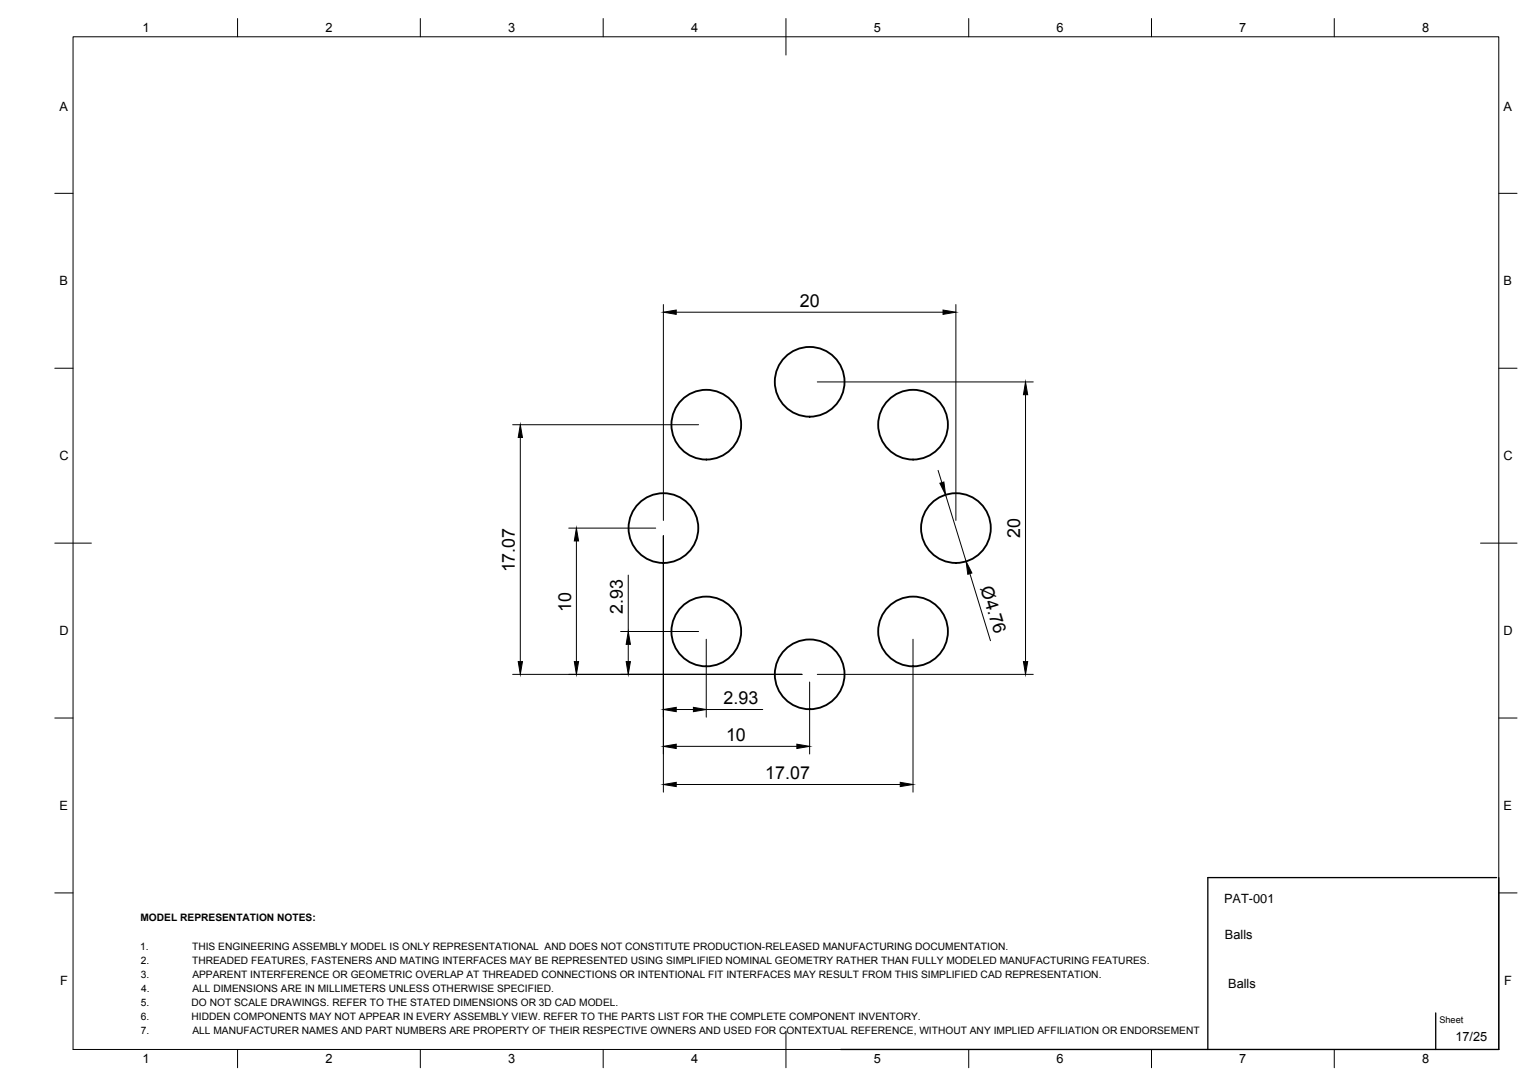
ISO-10303-21;
HEADER;
/* Generated by software containing ST-Developer
 * from STEP Tools, Inc. (www.steptools.com) 
 */

FILE_DESCRIPTION(
/* description */ ('PAT-001'),
/* implementation_level */ '2;1');

FILE_NAME(
/* name */ 'Balls.step',
/* time_stamp */ '2026-10-29T17:07:15-07:00',
/* author */ (''),
/* organization */ (''),
/* preprocessor_version */ 'ST-DEVELOPER v20.2',
/* originating_system */ 'Autodesk Translation Framework v15.17.0.0',
/* authorisation */ '');

FILE_SCHEMA (('AUTOMOTIVE_DESIGN { 1 0 10303 214 3 1 1 }'));
ENDSEC;

DATA;
#10=MECHANICAL_DESIGN_GEOMETRIC_PRESENTATION_REPRESENTATION('',(#380,#381,#382,#383,#384,#385,#386,#387),#9622);
#289=SPHERICAL_SURFACE('',#5611,0.23815);
#290=SPHERICAL_SURFACE('',#5613,0.23815);
#291=SPHERICAL_SURFACE('',#5615,0.23815);
#292=SPHERICAL_SURFACE('',#5617,0.23815);
#293=SPHERICAL_SURFACE('',#5619,0.23815);
#294=SPHERICAL_SURFACE('',#5621,0.23815);
#295=SPHERICAL_SURFACE('',#5623,0.23815);
#296=SPHERICAL_SURFACE('',#5625,0.23815);
#330=SHAPE_REPRESENTATION_RELATIONSHIP('SRR','None',#9754,#355);
#355=ADVANCED_BREP_SHAPE_REPRESENTATION('',(#413,#414,#415,#416,#417,#418,
#419,#420),#9603);
#380=STYLED_ITEM('',(#9962),#413);
#381=STYLED_ITEM('',(#9962),#414);
#382=STYLED_ITEM('',(#9962),#415);
#383=STYLED_ITEM('',(#9962),#416);
#384=STYLED_ITEM('',(#9962),#417);
#385=STYLED_ITEM('',(#9962),#418);
#386=STYLED_ITEM('',(#9962),#419);
#387=STYLED_ITEM('',(#9962),#420);
#413=MANIFOLD_SOLID_BREP('Body1',#5205);
#414=MANIFOLD_SOLID_BREP('Body2',#5206);
#415=MANIFOLD_SOLID_BREP('Body3',#5207);
#416=MANIFOLD_SOLID_BREP('Body4',#5208);
#417=MANIFOLD_SOLID_BREP('Body5',#5209);
#418=MANIFOLD_SOLID_BREP('Body6',#5210);
#419=MANIFOLD_SOLID_BREP('Body7',#5211);
#420=MANIFOLD_SOLID_BREP('Body8',#5212);
#758=FACE_OUTER_BOUND('',#1070,.T.);
#759=FACE_OUTER_BOUND('',#1071,.T.);
#760=FACE_OUTER_BOUND('',#1072,.T.);
#761=FACE_OUTER_BOUND('',#1073,.T.);
#762=FACE_OUTER_BOUND('',#1074,.T.);
#763=FACE_OUTER_BOUND('',#1075,.T.);
#764=FACE_OUTER_BOUND('',#1076,.T.);
#765=FACE_OUTER_BOUND('',#1077,.T.);
#1070=EDGE_LOOP('',(#3659,#3660));
#1071=EDGE_LOOP('',(#3661,#3662));
#1072=EDGE_LOOP('',(#3663,#3664));
#1073=EDGE_LOOP('',(#3665,#3666));
#1074=EDGE_LOOP('',(#3667,#3668));
#1075=EDGE_LOOP('',(#3669,#3670));
#1076=EDGE_LOOP('',(#3671,#3672));
#1077=EDGE_LOOP('',(#3673,#3674));
#2256=CIRCLE('',#5612,0.23815);
#2257=CIRCLE('',#5614,0.23815);
#2258=CIRCLE('',#5616,0.23815);
#2259=CIRCLE('',#5618,0.23815);
#2260=CIRCLE('',#5620,0.23815);
#2261=CIRCLE('',#5622,0.23815);
#2262=CIRCLE('',#5624,0.23815);
#2263=CIRCLE('',#5626,0.23815);
#2466=VERTEX_POINT('',#7880);
#2467=VERTEX_POINT('',#7881);
#2468=VERTEX_POINT('',#7884);
#2469=VERTEX_POINT('',#7885);
#2470=VERTEX_POINT('',#7888);
#2471=VERTEX_POINT('',#7889);
#2472=VERTEX_POINT('',#7892);
#2473=VERTEX_POINT('',#7893);
#2474=VERTEX_POINT('',#7896);
#2475=VERTEX_POINT('',#7897);
#2476=VERTEX_POINT('',#7900);
#2477=VERTEX_POINT('',#7901);
#2478=VERTEX_POINT('',#7904);
#2479=VERTEX_POINT('',#7905);
#2480=VERTEX_POINT('',#7908);
#2481=VERTEX_POINT('',#7909);
#2933=EDGE_CURVE('',#2466,#2467,#2256,.T.);
#2934=EDGE_CURVE('',#2468,#2469,#2257,.T.);
#2935=EDGE_CURVE('',#2470,#2471,#2258,.T.);
#2936=EDGE_CURVE('',#2472,#2473,#2259,.T.);
#2937=EDGE_CURVE('',#2474,#2475,#2260,.T.);
#2938=EDGE_CURVE('',#2476,#2477,#2261,.T.);
#2939=EDGE_CURVE('',#2478,#2479,#2262,.T.);
#2940=EDGE_CURVE('',#2480,#2481,#2263,.T.);
#3659=ORIENTED_EDGE('',*,*,#2933,.T.);
#3660=ORIENTED_EDGE('',*,*,#2933,.F.);
#3661=ORIENTED_EDGE('',*,*,#2934,.T.);
#3662=ORIENTED_EDGE('',*,*,#2934,.F.);
#3663=ORIENTED_EDGE('',*,*,#2935,.T.);
#3664=ORIENTED_EDGE('',*,*,#2935,.F.);
#3665=ORIENTED_EDGE('',*,*,#2936,.T.);
#3666=ORIENTED_EDGE('',*,*,#2936,.F.);
#3667=ORIENTED_EDGE('',*,*,#2937,.T.);
#3668=ORIENTED_EDGE('',*,*,#2937,.F.);
#3669=ORIENTED_EDGE('',*,*,#2938,.T.);
#3670=ORIENTED_EDGE('',*,*,#2938,.F.);
#3671=ORIENTED_EDGE('',*,*,#2939,.T.);
#3672=ORIENTED_EDGE('',*,*,#2939,.F.);
#3673=ORIENTED_EDGE('',*,*,#2940,.T.);
#3674=ORIENTED_EDGE('',*,*,#2940,.F.);
#4945=ADVANCED_FACE('',(#758),#289,.T.);
#4946=ADVANCED_FACE('',(#759),#290,.T.);
#4947=ADVANCED_FACE('',(#760),#291,.T.);
#4948=ADVANCED_FACE('',(#761),#292,.T.);
#4949=ADVANCED_FACE('',(#762),#293,.T.);
#4950=ADVANCED_FACE('',(#763),#294,.T.);
#4951=ADVANCED_FACE('',(#764),#295,.T.);
#4952=ADVANCED_FACE('',(#765),#296,.T.);
#5205=CLOSED_SHELL('',(#4945));
#5206=CLOSED_SHELL('',(#4946));
#5207=CLOSED_SHELL('',(#4947));
#5208=CLOSED_SHELL('',(#4948));
#5209=CLOSED_SHELL('',(#4949));
#5210=CLOSED_SHELL('',(#4950));
#5211=CLOSED_SHELL('',(#4951));
#5212=CLOSED_SHELL('',(#4952));
#5610=AXIS2_PLACEMENT_3D('',#7878,#6332,#6333);
#5611=AXIS2_PLACEMENT_3D('',#7879,#6334,#6335);
#5612=AXIS2_PLACEMENT_3D('',#7882,#6336,#6337);
#5613=AXIS2_PLACEMENT_3D('',#7883,#6338,#6339);
#5614=AXIS2_PLACEMENT_3D('',#7886,#6340,#6341);
#5615=AXIS2_PLACEMENT_3D('',#7887,#6342,#6343);
#5616=AXIS2_PLACEMENT_3D('',#7890,#6344,#6345);
#5617=AXIS2_PLACEMENT_3D('',#7891,#6346,#6347);
#5618=AXIS2_PLACEMENT_3D('',#7894,#6348,#6349);
#5619=AXIS2_PLACEMENT_3D('',#7895,#6350,#6351);
#5620=AXIS2_PLACEMENT_3D('',#7898,#6352,#6353);
#5621=AXIS2_PLACEMENT_3D('',#7899,#6354,#6355);
#5622=AXIS2_PLACEMENT_3D('',#7902,#6356,#6357);
#5623=AXIS2_PLACEMENT_3D('',#7903,#6358,#6359);
#5624=AXIS2_PLACEMENT_3D('',#7906,#6360,#6361);
#5625=AXIS2_PLACEMENT_3D('',#7907,#6362,#6363);
#5626=AXIS2_PLACEMENT_3D('',#7910,#6364,#6365);
#6332=DIRECTION('axis',(0.,0.,1.));
#6333=DIRECTION('refdir',(1.,0.,0.));
#6334=DIRECTION('center_axis',(0.,0.,1.));
#6335=DIRECTION('ref_axis',(1.,0.,0.));
#6336=DIRECTION('center_axis',(1.22464679914735E-16,-1.,0.));
#6337=DIRECTION('ref_axis',(-1.,-1.22464679914735E-16,0.));
#6338=DIRECTION('center_axis',(0.707106781186548,0.,0.707106781186548));
#6339=DIRECTION('ref_axis',(0.707106781186548,0.,-0.707106781186548));
#6340=DIRECTION('center_axis',(8.65956056235494E-17,-1.,-8.65956056235493E-17));
#6341=DIRECTION('ref_axis',(-0.707106781186547,-1.22464679914735E-16,0.707106781186547));
#6342=DIRECTION('center_axis',(1.,0.,0.));
#6343=DIRECTION('ref_axis',(6.12323399573676E-17,0.,-1.));
#6344=DIRECTION('center_axis',(7.49879891330929E-33,-1.,-1.22464679914735E-16));
#6345=DIRECTION('ref_axis',(-6.12323399573676E-17,-1.22464679914735E-16,
1.));
#6346=DIRECTION('center_axis',(0.707106781186548,0.,-0.707106781186548));
#6347=DIRECTION('ref_axis',(-0.707106781186548,0.,-0.707106781186548));
#6348=DIRECTION('center_axis',(-8.65956056235493E-17,-1.,-8.65956056235494E-17));
#6349=DIRECTION('ref_axis',(0.707106781186547,-1.22464679914735E-16,0.707106781186547));
#6350=DIRECTION('center_axis',(0.,0.,-1.));
#6351=DIRECTION('ref_axis',(-1.,0.,-1.22464679914735E-16));
#6352=DIRECTION('center_axis',(-1.22464679914735E-16,-1.,-1.49975978266186E-32));
#6353=DIRECTION('ref_axis',(1.,-1.22464679914735E-16,1.22464679914735E-16));
#6354=DIRECTION('center_axis',(-0.707106781186547,0.,-0.707106781186548));
#6355=DIRECTION('ref_axis',(-0.707106781186548,0.,0.707106781186547));
#6356=DIRECTION('center_axis',(-8.65956056235493E-17,-1.,8.65956056235493E-17));
#6357=DIRECTION('ref_axis',(0.707106781186548,-1.22464679914735E-16,-0.707106781186547));
#6358=DIRECTION('center_axis',(-1.,0.,0.));
#6359=DIRECTION('ref_axis',(-1.83697019872103E-16,0.,1.));
#6360=DIRECTION('center_axis',(-2.24963967399279E-32,-1.,1.22464679914735E-16));
#6361=DIRECTION('ref_axis',(1.83697019872103E-16,-1.22464679914735E-16,
-1.));
#6362=DIRECTION('center_axis',(-0.707106781186548,0.,0.707106781186548));
#6363=DIRECTION('ref_axis',(0.707106781186547,0.,0.707106781186548));
#6364=DIRECTION('center_axis',(8.65956056235493E-17,-1.,8.65956056235493E-17));
#6365=DIRECTION('ref_axis',(-0.707106781186547,-1.22464679914735E-16,-0.707106781186548));
#7878=CARTESIAN_POINT('',(0.,0.,0.));
#7879=CARTESIAN_POINT('Origin',(1.,0.,0.));
#7880=CARTESIAN_POINT('',(1.,-1.78583896120461E-33,0.23815));
#7881=CARTESIAN_POINT('',(1.,-1.78583896120461E-33,-0.23815));
#7882=CARTESIAN_POINT('Origin',(1.,0.,0.));
#7883=CARTESIAN_POINT('Origin',(0.707106781186548,0.,-0.707106781186547));
#7884=CARTESIAN_POINT('',(0.875504261126124,-1.78583896120461E-33,-0.538709301246971));
#7885=CARTESIAN_POINT('',(0.538709301246971,-1.78583896120461E-33,-0.875504261126124));
#7886=CARTESIAN_POINT('Origin',(0.707106781186548,0.,-0.707106781186547));
#7887=CARTESIAN_POINT('Origin',(6.12323399573677E-17,0.,-1.));
#7888=CARTESIAN_POINT('',(0.23815,-1.78583896120461E-33,-1.));
#7889=CARTESIAN_POINT('',(-0.23815,-1.78583896120461E-33,-1.));
#7890=CARTESIAN_POINT('Origin',(6.12323399573677E-17,0.,-1.));
#7891=CARTESIAN_POINT('Origin',(-0.707106781186547,0.,-0.707106781186548));
#7892=CARTESIAN_POINT('',(-0.538709301246971,-1.78583896120461E-33,-0.875504261126124));
#7893=CARTESIAN_POINT('',(-0.875504261126124,-1.78583896120461E-33,-0.538709301246971));
#7894=CARTESIAN_POINT('Origin',(-0.707106781186547,0.,-0.707106781186548));
#7895=CARTESIAN_POINT('Origin',(-1.,0.,-1.22464679914735E-16));
#7896=CARTESIAN_POINT('',(-1.,-1.78583896120461E-33,-0.23815));
#7897=CARTESIAN_POINT('',(-1.,-1.78583896120461E-33,0.23815));
#7898=CARTESIAN_POINT('Origin',(-1.,0.,-1.22464679914735E-16));
#7899=CARTESIAN_POINT('Origin',(-0.707106781186548,0.,0.707106781186547));
#7900=CARTESIAN_POINT('',(-0.875504261126124,-7.94881478324376E-33,0.538709301246971));
#7901=CARTESIAN_POINT('',(-0.538709301246971,4.37713686083455E-33,0.875504261126124));
#7902=CARTESIAN_POINT('Origin',(-0.707106781186548,0.,0.707106781186547));
#7903=CARTESIAN_POINT('Origin',(-1.83697019872103E-16,0.,1.));
#7904=CARTESIAN_POINT('',(-0.23815,-1.78583896120461E-33,1.));
#7905=CARTESIAN_POINT('',(0.23815,-1.78583896120461E-33,1.));
#7906=CARTESIAN_POINT('Origin',(-1.83697019872103E-16,0.,1.));
#7907=CARTESIAN_POINT('Origin',(0.707106781186547,0.,0.707106781186548));
#7908=CARTESIAN_POINT('',(0.538709301246971,-4.86732687222419E-33,0.875504261126124));
#7909=CARTESIAN_POINT('',(0.875504261126124,1.29564894981497E-33,0.538709301246971));
#7910=CARTESIAN_POINT('Origin',(0.707106781186547,0.,0.707106781186548));
#9573=UNCERTAINTY_MEASURE_WITH_UNIT(LENGTH_MEASURE(0.001),#9623,
'DISTANCE_ACCURACY_VALUE',
'Maximum model space distance between geometric entities at asserted c
onnectivities');
#9592=UNCERTAINTY_MEASURE_WITH_UNIT(LENGTH_MEASURE(0.001),#9623,
'DISTANCE_ACCURACY_VALUE',
'Maximum model space distance between geometric entities at asserted c
onnectivities');
#9603=(
GEOMETRIC_REPRESENTATION_CONTEXT(3)
GLOBAL_UNCERTAINTY_ASSIGNED_CONTEXT((#9573))
GLOBAL_UNIT_ASSIGNED_CONTEXT((#9623,#9625,#9626))
REPRESENTATION_CONTEXT('','3D')
);
#9622=(
GEOMETRIC_REPRESENTATION_CONTEXT(3)
GLOBAL_UNCERTAINTY_ASSIGNED_CONTEXT((#9592))
GLOBAL_UNIT_ASSIGNED_CONTEXT((#9623,#9625,#9626))
REPRESENTATION_CONTEXT('','3D')
);
#9623=(
LENGTH_UNIT()
NAMED_UNIT(*)
SI_UNIT(.CENTI.,.METRE.)
);
#9625=(
NAMED_UNIT(*)
PLANE_ANGLE_UNIT()
SI_UNIT($,.RADIAN.)
);
#9626=(
NAMED_UNIT(*)
SI_UNIT($,.STERADIAN.)
SOLID_ANGLE_UNIT()
);
#9637=SHAPE_DEFINITION_REPRESENTATION(#9666,#9754);
#9666=PRODUCT_DEFINITION_SHAPE('',$,#9784);
#9754=SHAPE_REPRESENTATION('',(#5610),#9603);
#9773=PRODUCT_DEFINITION_CONTEXT('part definition',#9862,'design');
#9784=PRODUCT_DEFINITION('Balls','Balls',#9813,#9773);
#9813=PRODUCT_DEFINITION_FORMATION('',$,#9874);
#9862=APPLICATION_CONTEXT(
'Core Data for Automotive Mechanical Design Process');
#9863=PRODUCT_CONTEXT('part definition',#9862,'mechanical');
#9874=PRODUCT('Balls','Balls','Balls',(#9863));
#9956=COLOUR_RGB('Grey',0.48,0.52,0.57);
#9957=FILL_AREA_STYLE_COLOUR('',#9956);
#9958=FILL_AREA_STYLE('',(#9957));
#9959=SURFACE_STYLE_FILL_AREA(#9958);
#9960=SURFACE_SIDE_STYLE('',(#9959));
#9961=SURFACE_STYLE_USAGE(.BOTH.,#9960);
#9962=PRESENTATION_STYLE_ASSIGNMENT((#9961));
ENDSEC;
END-ISO-10303-21;
